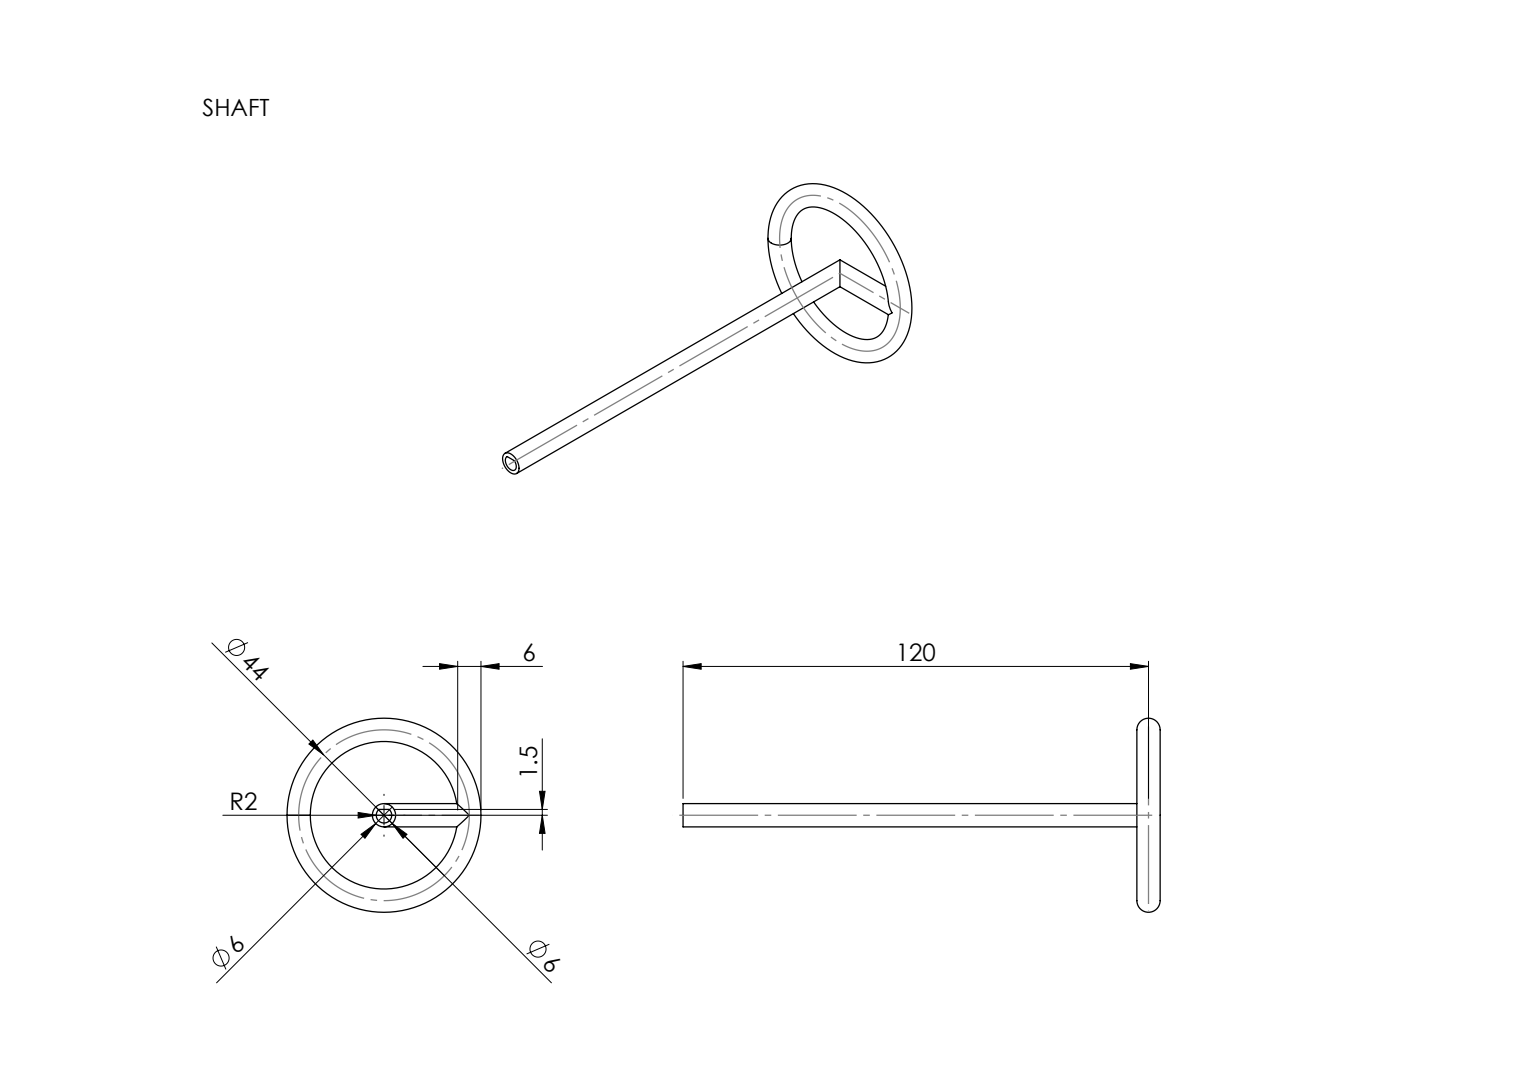
ISO-10303-21;
HEADER;
FILE_DESCRIPTION (('STEP AP214'),
    '1' );
FILE_NAME ('shaft.step',
    '2026-10-08T15:02:10',
    ( '' ),
    ( '' ),
    'SwSTEP 2.0',
    'SolidWorks 2026',
    '' );
FILE_SCHEMA (( 'AUTOMOTIVE_DESIGN' ));
ENDSEC;

DATA;
#29=AXIS2_PLACEMENT_3D ( 'NONE', #18064, #14475, #11199 ) ;
#50=SURFACE_SIDE_STYLE ('',( #17385 ) ) ;
#60=ORIENTED_EDGE ( 'NONE', *, *, #7917, .F. ) ;
#89=CARTESIAN_POINT ( 'NONE',  ( 18.76166303929371537, -3.000000000000002665, -225.0000000000001990 ) ) ;
#116=DIRECTION ( 'NONE',  ( -1.000000000000000000, 0.000000000000000000, 0.000000000000000000 ) ) ;
#168=SURFACE_STYLE_USAGE ( .BOTH. , #50 ) ;
#218=ORIENTED_EDGE ( 'NONE', *, *, #19552, .T. ) ;
#247=CARTESIAN_POINT ( 'NONE',  ( 0.000000000000000000, 0.000000000000000000, -120.0000000000000142 ) ) ;
#414=ORIENTED_EDGE ( 'NONE', *, *, #15901, .T. ) ;
#621=B_SPLINE_CURVE_WITH_KNOTS ( 'NONE', 3,
 ( #8461, #18585, #1249, #11827, #16893, #8123, #21829, #13288, #15329, #18471, #10030, #3033, #3147, #1359, #8232, #15102, #1467, #8343, #15214, #6763, #13633, #22059 ),
 .UNSPECIFIED., .F., .F.,
 ( 4, 2, 2, 2, 2, 2, 2, 2, 2, 2, 4 ),
 ( 0.005800309973860217315, 0.006162931802046735415, 0.006525553630233253515, 0.006888175458419771614, 0.007250797286606289714, 0.007976040942979321577, 0.008701284599352352572, 0.01015177191209841456, 0.01087701556847144729, 0.01123963739665796366, 0.01160225922484448176 ),
 .UNSPECIFIED. ) ;
#691=DIRECTION ( 'NONE',  ( -2.891205793294678696E-17, 0.000000000000000000, -1.000000000000000000 ) ) ;
#722=VERTEX_POINT ( 'NONE', #4541 ) ;
#733=PRODUCT_CONTEXT ( 'NONE', #18778, 'mechanical' ) ;
#748=DIRECTION ( 'NONE',  ( -0.000000000000000000, -1.000000000000000000, 0.000000000000000000 ) ) ;
#799=CARTESIAN_POINT ( 'NONE',  ( 18.92955364685790798, 2.856280672885327832, -224.0526243428037105 ) ) ;
#867=FACE_OUTER_BOUND ( 'NONE', #7455, .T. ) ;
#876=ADVANCED_FACE ( 'NONE', ( #9133 ), #19112, .T. ) ;
#940=DIRECTION ( 'NONE',  ( 1.000000000000000000, 0.000000000000000000, 0.000000000000000000 ) ) ;
#951=CARTESIAN_POINT ( 'NONE',  ( -1.322875655532295136, 1.500000000000000000, -105.0000000000000142 ) ) ;
#991=SHAPE_REPRESENTATION_RELATIONSHIP ( 'NONE' , 'NONE' ,  #6134, #7772 ) ;
#1072=DIRECTION ( 'NONE',  ( -2.891205793294678696E-17, 0.000000000000000000, -1.000000000000000000 ) ) ;
#1087=DIRECTION ( 'NONE',  ( -1.000000000000000000, 0.000000000000000000, 2.891205793294678696E-17 ) ) ;
#1143=AXIS2_PLACEMENT_3D ( 'NONE', #18620, #15780, #13440 ) ;
#1193=CARTESIAN_POINT ( 'NONE',  ( -3.400000000000003908, 0.000000000000000000, -224.9999999999999716 ) ) ;
#1202=ORIENTED_EDGE ( 'NONE', *, *, #20807, .F. ) ;
#1215=CARTESIAN_POINT ( 'NONE',  ( 19.81239090451984097, -2.079411191919079638, -222.8294590615037123 ) ) ;
#1249=CARTESIAN_POINT ( 'NONE',  ( 18.77064933249683065, 2.992341472042430173, -225.2461773443920663 ) ) ;
#1297=DIRECTION ( 'NONE',  ( -2.891205793294678696E-17, 0.000000000000000000, -1.000000000000000000 ) ) ;
#1304=CYLINDRICAL_SURFACE ( 'NONE', #3314, 3.000000000000002665 ) ;
#1319=CARTESIAN_POINT ( 'NONE',  ( -2.775557561562891351E-14, 0.000000000000000000, -105.0000000000000142 ) ) ;
#1327=CARTESIAN_POINT ( 'NONE',  ( 22.00000000000000000, 0.000000000000000000, -221.9999999999999716 ) ) ;
#1359=CARTESIAN_POINT ( 'NONE',  ( 20.28602808787860567, 1.649471991126377768, -227.5337793182429493 ) ) ;
#1463=FACE_OUTER_BOUND ( 'NONE', #17228, .T. ) ;
#1467=CARTESIAN_POINT ( 'NONE',  ( 21.30611872263677498, 0.6836234283288439295, -227.9261315426025760 ) ) ;
#1469=( NAMED_UNIT ( * ) PLANE_ANGLE_UNIT ( ) SI_UNIT ( $, .RADIAN. ) );
#1480=DIRECTION ( 'NONE',  ( -6.123233995736766036E-17, 0.000000000000000000, 1.000000000000000000 ) ) ;
#1549=PLANE ( 'NONE',  #9838 ) ;
#1587=SURFACE_STYLE_FILL_AREA ( #3257 ) ;
#1634=( LENGTH_UNIT ( ) NAMED_UNIT ( * ) SI_UNIT ( .MILLI., .METRE. ) );
#1673=ORIENTED_EDGE ( 'NONE', *, *, #20807, .T. ) ;
#1678=ORIENTED_EDGE ( 'NONE', *, *, #12038, .T. ) ;
#1923=CARTESIAN_POINT ( 'NONE',  ( -3.000000000000034195, 6.000000000000006217, -227.9999999999999716 ) ) ;
#1949=EDGE_CURVE ( 'NONE', #722, #21305, #10868, .T. ) ;
#1961=( GEOMETRIC_REPRESENTATION_CONTEXT ( 3 ) GLOBAL_UNCERTAINTY_ASSIGNED_CONTEXT ( ( #19989 ) ) GLOBAL_UNIT_ASSIGNED_CONTEXT ( ( #1634, #15705, #7260 ) ) REPRESENTATION_CONTEXT ( 'NONE', 'WORKASPACE' ) );
#2075=DIRECTION ( 'NONE',  ( -1.000000000000000000, 0.000000000000000000, 0.000000000000000000 ) ) ;
#2085=CARTESIAN_POINT ( 'NONE',  ( 2.000000000000000000, 0.000000000000000000, -120.0000000000000142 ) ) ;
#2086=ORIENTED_EDGE ( 'NONE', *, *, #21351, .F. ) ;
#2168=CLOSED_SHELL ( 'NONE', ( #876, #15317, #2802, #6387, #3276, #20231, #8918, #6260, #11075, #12311, #16542, #17405, #7759, #13941 ) ) ;
#2200=ORIENTED_EDGE ( 'NONE', *, *, #7776, .F. ) ;
#2204=DIRECTION ( 'NONE',  ( -1.000000000000000000, -1.224646799147353454E-16, 0.000000000000000000 ) ) ;
#2259=AXIS2_PLACEMENT_3D ( 'NONE', #13081, #18367, #16564 ) ;
#2343=DIRECTION ( 'NONE',  ( -1.000000000000000000, 0.000000000000000000, 0.000000000000000000 ) ) ;
#2453=DIRECTION ( 'NONE',  ( 1.000000000000000000, 0.000000000000000000, 0.000000000000000000 ) ) ;
#2484=CARTESIAN_POINT ( 'NONE',  ( 19.66316721362388975, 2.213178807039652973, -222.9648072419893765 ) ) ;
#2565=DIRECTION ( 'NONE',  ( -1.000000000000000000, 0.000000000000000000, 0.000000000000000000 ) ) ;
#2593=FACE_OUTER_BOUND ( 'NONE', #12316, .T. ) ;
#2604=CARTESIAN_POINT ( 'NONE',  ( 1.322875655532295358, 1.500000000000000000, -105.0000000000000142 ) ) ;
#2609=VECTOR ( 'NONE', #2075, 1000.000000000000000 ) ;
#2707=DIRECTION ( 'NONE',  ( 1.000000000000000000, 0.000000000000000000, 0.000000000000000000 ) ) ;
#2762=VERTEX_POINT ( 'NONE', #21336 ) ;
#2802=ADVANCED_FACE ( 'NONE', ( #867 ), #4621, .T. ) ;
#2874=ORIENTED_EDGE ( 'NONE', *, *, #19438, .T. ) ;
#2885=CARTESIAN_POINT ( 'NONE',  ( 19.08116649778970952, -2.725278401796281447, -223.7411956188273621 ) ) ;
#2965=VERTEX_POINT ( 'NONE', #19869 ) ;
#2978=CARTESIAN_POINT ( 'NONE',  ( 22.00000000000000000, 6.162975822039154730E-30, -228.0000000000000000 ) ) ;
#3000=CARTESIAN_POINT ( 'NONE',  ( 19.24993070808567097, -2.578473320807608715, -223.4513235704932299 ) ) ;
#3004=CARTESIAN_POINT ( 'NONE',  ( 21.82657638218437057, -0.1729100361068852398, -227.9962408443968798 ) ) ;
#3033=CARTESIAN_POINT ( 'NONE',  ( 19.66230024959844513, 2.213945732971074332, -227.0341823791074773 ) ) ;
#3102=CARTESIAN_POINT ( 'NONE',  ( 0.000000000000000000, 0.000000000000000000, -120.0000000000000142 ) ) ;
#3147=CARTESIAN_POINT ( 'NONE',  ( 19.81239090451986939, 2.079411191919064983, -227.1705409384963161 ) ) ;
#3190=ORIENTED_EDGE ( 'NONE', *, *, #9938, .T. ) ;
#3194=DIRECTION ( 'NONE',  ( 1.000000000000000000, 0.000000000000000000, 0.000000000000000000 ) ) ;
#3257=FILL_AREA_STYLE ('',( #6873 ) ) ;
#3276=ADVANCED_FACE ( 'NONE', ( #5013 ), #15389, .F. ) ;
#3314=AXIS2_PLACEMENT_3D ( 'NONE', #1193, #18305, #11216 ) ;
#3339=CARTESIAN_POINT ( 'NONE',  ( 19.81538647100171957, -2.076704763782542429, -227.1730004250662773 ) ) ;
#3371=PRESENTATION_STYLE_ASSIGNMENT (( #21940 ) ) ;
#3386=COLOUR_RGB ( '', 0.31764706, 0.68627451, 0.89019608) ;
#3449=CARTESIAN_POINT ( 'NONE',  ( 0.000000000000000000, 0.000000000000000000, -120.0000000000000142 ) ) ;
#3542=ORIENTED_EDGE ( 'NONE', *, *, #3964, .T. ) ;
#3565=EDGE_CURVE ( 'NONE', #8742, #7031, #18647, .T. ) ;
#3572=VERTEX_POINT ( 'NONE', #6600 ) ;
#3663=DIRECTION ( 'NONE',  ( 0.000000000000000000, 0.000000000000000000, -1.000000000000000000 ) ) ;
#3669=CARTESIAN_POINT ( 'NONE',  ( 19.25067847059915849, -2.577822808762990636, -226.5499581033751895 ) ) ;
#3694=DIRECTION ( 'NONE',  ( 1.000000000000000000, 0.000000000000000000, 0.000000000000000000 ) ) ;
#3750=TOROIDAL_SURFACE ( 'NONE', #8452, 22.00000000000000711, 2.999999999999999112 ) ;
#3775=VECTOR ( 'NONE', #17147, 1000.000000000000000 ) ;
#3788=CARTESIAN_POINT ( 'NONE',  ( 18.83061188870375702, -2.941116900365129183, -225.6031553348211958 ) ) ;
#3830=DIRECTION ( 'NONE',  ( 1.000000000000000000, 0.000000000000000000, 0.000000000000000000 ) ) ;
#3964=EDGE_CURVE ( 'NONE', #17015, #11981, #7055, .T. ) ;
#4056=CIRCLE ( 'NONE', #2259, 2.000000000000000000 ) ;
#4072=AXIS2_PLACEMENT_3D ( 'NONE', #9335, #12708, #16635 ) ;
#4111=ORIENTED_EDGE ( 'NONE', *, *, #13596, .T. ) ;
#4126=ORIENTED_EDGE ( 'NONE', *, *, #11026, .T. ) ;
#4175=VECTOR ( 'NONE', #20468, 1000.000000000000000 ) ;
#4250=CYLINDRICAL_SURFACE ( 'NONE', #8056, 3.000000000000002665 ) ;
#4307=ORIENTED_EDGE ( 'NONE', *, *, #10113, .F. ) ;
#4332=FACE_OUTER_BOUND ( 'NONE', #8944, .T. ) ;
#4364=ORIENTED_EDGE ( 'NONE', *, *, #8228, .T. ) ;
#4443=EDGE_CURVE ( 'NONE', #17126, #4726, #6051, .T. ) ;
#4448=ORIENTED_EDGE ( 'NONE', *, *, #14092, .F. ) ;
#4452=ORIENTED_EDGE ( 'NONE', *, *, #1949, .F. ) ;
#4541=CARTESIAN_POINT ( 'NONE',  ( 24.99999999999999645, 3.061616997868383437E-15, -224.9999999999999716 ) ) ;
#4570=ORIENTED_EDGE ( 'NONE', *, *, #14092, .T. ) ;
#4621=TOROIDAL_SURFACE ( 'NONE', #6424, 22.00000000000000711, 2.999999999999999112 ) ;
#4688=CARTESIAN_POINT ( 'NONE',  ( 21.82670294635402897, -0.1727854921979527503, -222.0037445873432205 ) ) ;
#4726=VERTEX_POINT ( 'NONE', #951 ) ;
#4808=DIRECTION ( 'NONE',  ( -0.000000000000000000, -0.000000000000000000, 1.000000000000000000 ) ) ;
#4818=CIRCLE ( 'NONE', #9908, 2.999999999999999112 ) ;
#4840=( NAMED_UNIT ( * ) SI_UNIT ( $, .STERADIAN. ) SOLID_ANGLE_UNIT ( ) );
#4888=CARTESIAN_POINT ( 'NONE',  ( -6.938893903907228378E-15, 0.000000000000000000, -224.9999999999999716 ) ) ;
#5007=EDGE_LOOP ( 'NONE', ( #11084, #5257, #4307, #6425 ) ) ;
#5013=FACE_OUTER_BOUND ( 'NONE', #11808, .T. ) ;
#5025=DIRECTION ( 'NONE',  ( -0.000000000000000000, -0.000000000000000000, 1.000000000000000000 ) ) ;
#5030=CARTESIAN_POINT ( 'NONE',  ( 20.29114891157122358, -1.643118446426441892, -227.5163857825534421 ) ) ;
#5035=ORIENTED_EDGE ( 'NONE', *, *, #17379, .T. ) ;
#5060=( LENGTH_UNIT ( ) NAMED_UNIT ( * ) SI_UNIT ( .MILLI., .METRE. ) );
#5234=ORIENTED_EDGE ( 'NONE', *, *, #19552, .F. ) ;
#5237=LINE ( 'NONE', #13472, #19455 ) ;
#5257=ORIENTED_EDGE ( 'NONE', *, *, #13812, .T. ) ;
#5364=EDGE_LOOP ( 'NONE', ( #11204, #4448, #4126, #60 ) ) ;
#5375=EDGE_CURVE ( 'NONE', #18785, #9979, #5237, .T. ) ;
#5477=CARTESIAN_POINT ( 'NONE',  ( -6.938893903907228378E-15, 0.000000000000000000, -224.9999999999999716 ) ) ;
#5520=FACE_OUTER_BOUND ( 'NONE', #22180, .T. ) ;
#5555=VERTEX_POINT ( 'NONE', #10208 ) ;
#5604=VERTEX_POINT ( 'NONE', #16961 ) ;
#5679=DIRECTION ( 'NONE',  ( -0.000000000000000000, -0.000000000000000000, 1.000000000000000000 ) ) ;
#5701=DIRECTION ( 'NONE',  ( -1.000000000000000000, 0.000000000000000000, 0.000000000000000000 ) ) ;
#5718=CARTESIAN_POINT ( 'NONE',  ( 0.000000000000000000, 0.000000000000000000, -120.0000000000000142 ) ) ;
#5818=CARTESIAN_POINT ( 'NONE',  ( -6.938893903907228378E-15, 0.000000000000000000, -224.9999999999999716 ) ) ;
#5854=AXIS2_PLACEMENT_3D ( 'NONE', #20104, #4808, #20213 ) ;
#5860=CARTESIAN_POINT ( 'NONE',  ( -6.938893903907228378E-15, 0.000000000000000000, -224.9999999999999716 ) ) ;
#5881=ORIENTED_EDGE ( 'NONE', *, *, #3565, .F. ) ;
#5925=ORIENTED_EDGE ( 'NONE', *, *, #8488, .T. ) ;
#5975=AXIS2_PLACEMENT_3D ( 'NONE', #12852, #16554, #20027 ) ;
#6051=CIRCLE ( 'NONE', #19700, 2.000000000000000000 ) ;
#6082=CARTESIAN_POINT ( 'NONE',  ( 19.81538647100178707, 2.076704763782484253, -222.8269995749336658 ) ) ;
#6130=CARTESIAN_POINT ( 'NONE',  ( -22.00000000000001421, 0.000000000000000000, -224.9999999999999716 ) ) ;
#6134=SHAPE_REPRESENTATION ( 'shaft', ( #6677 ), #8503 ) ;
#6240=CIRCLE ( 'NONE', #9120, 2.000000000000000000 ) ;
#6246=DIRECTION ( 'NONE',  ( -2.891205793294678696E-17, 0.000000000000000000, -1.000000000000000000 ) ) ;
#6260=ADVANCED_FACE ( 'NONE', ( #7607, #9625 ), #21757, .T. ) ;
#6325=ORIENTED_EDGE ( 'NONE', *, *, #15901, .F. ) ;
#6327=ORIENTED_EDGE ( 'NONE', *, *, #11715, .T. ) ;
#6383=CARTESIAN_POINT ( 'NONE',  ( 21.56647080447662290, -0.4294288297056042536, -222.0296485764623640 ) ) ;
#6387=ADVANCED_FACE ( 'NONE', ( #5520 ), #12398, .F. ) ;
#6424=AXIS2_PLACEMENT_3D ( 'NONE', #5818, #19543, #1087 ) ;
#6425=ORIENTED_EDGE ( 'NONE', *, *, #11026, .F. ) ;
#6487=DIRECTION ( 'NONE',  ( -1.000000000000000000, 0.000000000000000000, 0.000000000000000000 ) ) ;
#6529=CARTESIAN_POINT ( 'NONE',  ( 2.999999999999972466, -6.000000000000006217, -221.9999999999999716 ) ) ;
#6600=CARTESIAN_POINT ( 'NONE',  ( 22.00000000000000000, 0.000000000000000000, -221.9999999999999716 ) ) ;
#6613=CARTESIAN_POINT ( 'NONE',  ( -2.000000000000000000, 2.449293598294706414E-16, -120.0000000000000142 ) ) ;
#6614=CARTESIAN_POINT ( 'NONE',  ( 19.02965008953347237, -2.769875716686367007, -223.8421603075141491 ) ) ;
#6619=CARTESIAN_POINT ( 'NONE',  ( -2.775557561562891351E-14, 0.000000000000000000, -105.0000000000000142 ) ) ;
#6648=CARTESIAN_POINT ( 'NONE',  ( -3.400000000000003908, 0.000000000000000000, -227.9999999999999716 ) ) ;
#6677=AXIS2_PLACEMENT_3D ( 'NONE', #18028, #16226, #2707 ) ;
#6711=AXIS2_PLACEMENT_3D ( 'NONE', #5860, #691, #14761 ) ;
#6732=CARTESIAN_POINT ( 'NONE',  ( 18.93769218002321253, -2.849225658158391461, -224.0541049803088356 ) ) ;
#6763=CARTESIAN_POINT ( 'NONE',  ( 21.82670294635401831, 0.1727854921979470326, -227.9962554126566943 ) ) ;
#6868=DIRECTION ( 'NONE',  ( -2.891205793294678696E-17, 0.000000000000000000, -1.000000000000000000 ) ) ;
#6873=FILL_AREA_STYLE_COLOUR ( '', #15337 ) ;
#6886=CARTESIAN_POINT ( 'NONE',  ( 2.999999999999970690, 6.000000000000006217, -221.9999999999999716 ) ) ;
#6941=ORIENTED_EDGE ( 'NONE', *, *, #11715, .F. ) ;
#7031=VERTEX_POINT ( 'NONE', #9414 ) ;
#7055=LINE ( 'NONE', #2085, #7143 ) ;
#7143=VECTOR ( 'NONE', #5679, 1000.000000000000000 ) ;
#7260=( NAMED_UNIT ( * ) SI_UNIT ( $, .STERADIAN. ) SOLID_ANGLE_UNIT ( ) );
#7314=CIRCLE ( 'NONE', #16629, 19.00000000000000711 ) ;
#7455=EDGE_LOOP ( 'NONE', ( #14480, #15948, #5925, #2200, #9544 ) ) ;
#7567=EDGE_CURVE ( 'NONE', #7956, #5604, #15692, .T. ) ;
#7607=FACE_BOUND ( 'NONE', #14199, .T. ) ;
#7679=CARTESIAN_POINT ( 'NONE',  ( 18.83061188870378544, 2.941116900365108311, -224.3968446651786337 ) ) ;
#7688=CIRCLE ( 'NONE', #4072, 2.999999999999999112 ) ;
#7715=DIRECTION ( 'NONE',  ( 1.000000000000000000, 0.000000000000000000, 0.000000000000000000 ) ) ;
#7724=ORIENTED_EDGE ( 'NONE', *, *, #21351, .T. ) ;
#7759=ADVANCED_FACE ( 'NONE', ( #2593 ), #7901, .F. ) ;
#7772=ADVANCED_BREP_SHAPE_REPRESENTATION ( '', ( #14254, #6677 ), #8503 ) ;
#7776=EDGE_CURVE ( 'NONE', #3572, #5555, #19145, .T. ) ;
#7793=CARTESIAN_POINT ( 'NONE',  ( 19.38023697009521840, 2.464236985537108904, -223.2772968702357730 ) ) ;
#7795=CARTESIAN_POINT ( 'NONE',  ( -3.000000000000030198, 0.000000000000000000, -105.0000000000000142 ) ) ;
#7817=DIRECTION ( 'NONE',  ( 6.123233995736766036E-17, -0.000000000000000000, -1.000000000000000000 ) ) ;
#7896=EDGE_LOOP ( 'NONE', ( #4570, #14262 ) ) ;
#7901=PLANE ( 'NONE',  #5975 ) ;
#7917=EDGE_CURVE ( 'NONE', #2965, #2762, #20795, .T. ) ;
#7956=VERTEX_POINT ( 'NONE', #20244 ) ;
#7975=FACE_OUTER_BOUND ( 'NONE', #19124, .T. ) ;
#8009=CARTESIAN_POINT ( 'NONE',  ( 21.30903826138442270, 0.6807850236355362794, -222.0732863424555035 ) ) ;
#8056=AXIS2_PLACEMENT_3D ( 'NONE', #18326, #2453, #14732 ) ;
#8085=UNCERTAINTY_MEASURE_WITH_UNIT (LENGTH_MEASURE( 1.000000000000000082E-05 ), #5060, 'distance_accuracy_value', 'NONE');
#8090=CARTESIAN_POINT ( 'NONE',  ( 21.30611872263680695, -0.6836234283288118441, -222.0738684573972819 ) ) ;
#8111=VECTOR ( 'NONE', #3694, 1000.000000000000000 ) ;
#8123=CARTESIAN_POINT ( 'NONE',  ( 18.89697753402894875, 2.884212079946345320, -225.8338386031039988 ) ) ;
#8149=CARTESIAN_POINT ( 'NONE',  ( -25.00000000000001066, 0.000000000000000000, -224.9999999999999716 ) ) ;
#8177=EDGE_CURVE ( 'NONE', #5555, #9014, #621, .T. ) ;
#8198=CARTESIAN_POINT ( 'NONE',  ( 2.000000000000000000, 0.000000000000000000, -120.0000000000000142 ) ) ;
#8228=EDGE_CURVE ( 'NONE', #2762, #9014, #20357, .T. ) ;
#8232=CARTESIAN_POINT ( 'NONE',  ( 20.61940245508341363, 1.339931705218432079, -227.7063352817440318 ) ) ;
#8234=( NAMED_UNIT ( * ) PLANE_ANGLE_UNIT ( ) SI_UNIT ( $, .RADIAN. ) );
#8259=LINE ( 'NONE', #16921, #3775 ) ;
#8288=EDGE_CURVE ( 'NONE', #5604, #21305, #10669, .T. ) ;
#8302=DIRECTION ( 'NONE',  ( -2.891205793294678696E-17, 0.000000000000000000, -1.000000000000000000 ) ) ;
#8343=CARTESIAN_POINT ( 'NONE',  ( 21.56647080447661224, 0.4294288297056144676, -227.9703514235376076 ) ) ;
#8413=ORIENTED_EDGE ( 'NONE', *, *, #1949, .T. ) ;
#8430=FACE_OUTER_BOUND ( 'NONE', #19282, .T. ) ;
#8452=AXIS2_PLACEMENT_3D ( 'NONE', #4888, #1072, #19966 ) ;
#8461=CARTESIAN_POINT ( 'NONE',  ( 18.76166303929371537, 3.000000000000002665, -224.9999999999997442 ) ) ;
#8488=EDGE_CURVE ( 'NONE', #5604, #5555, #7314, .T. ) ;
#8503=( GEOMETRIC_REPRESENTATION_CONTEXT ( 3 ) GLOBAL_UNCERTAINTY_ASSIGNED_CONTEXT ( ( #8085 ) ) GLOBAL_UNIT_ASSIGNED_CONTEXT ( ( #5060, #1469, #11937 ) ) REPRESENTATION_CONTEXT ( 'NONE', 'WORKASPACE' ) );
#8742=VERTEX_POINT ( 'NONE', #12799 ) ;
#8918=ADVANCED_FACE ( 'NONE', ( #4332 ), #1304, .T. ) ;
#8944=EDGE_LOOP ( 'NONE', ( #12143, #414, #16206, #20787, #17415 ) ) ;
#9014=VERTEX_POINT ( 'NONE', #2978 ) ;
#9120=AXIS2_PLACEMENT_3D ( 'NONE', #5718, #19114, #2343 ) ;
#9133=FACE_OUTER_BOUND ( 'NONE', #18914, .T. ) ;
#9165=ORIENTED_EDGE ( 'NONE', *, *, #4443, .F. ) ;
#9335=CARTESIAN_POINT ( 'NONE',  ( 22.00000000000000000, 2.694222958124177598E-15, -224.9999999999999716 ) ) ;
#9414=CARTESIAN_POINT ( 'NONE',  ( -1.322875655532295136, 1.500000000000000000, -120.0000000000000142 ) ) ;
#9476=CARTESIAN_POINT ( 'NONE',  ( 20.12875910279714020, 1.792218354162522953, -222.5869962921167655 ) ) ;
#9544=ORIENTED_EDGE ( 'NONE', *, *, #13072, .T. ) ;
#9568=ORIENTED_EDGE ( 'NONE', *, *, #12948, .F. ) ;
#9625=FACE_OUTER_BOUND ( 'NONE', #7896, .T. ) ;
#9695=LINE ( 'NONE', #7795, #19957 ) ;
#9838=AXIS2_PLACEMENT_3D ( 'NONE', #3449, #3663, #17191 ) ;
#9883=CARTESIAN_POINT ( 'NONE',  ( 19.66230024959842382, -2.213945732971099201, -222.9658176208924942 ) ) ;
#9887=CARTESIAN_POINT ( 'NONE',  ( 21.30903826138435875, -0.6807850236355832418, -227.9267136575444397 ) ) ;
#9891=TOROIDAL_SURFACE ( 'NONE', #12418, 22.00000000000000711, 2.999999999999999112 ) ;
#9908=AXIS2_PLACEMENT_3D ( 'NONE', #12017, #12353, #2204 ) ;
#9938=EDGE_CURVE ( 'NONE', #9979, #11981, #4056, .T. ) ;
#9979=VERTEX_POINT ( 'NONE', #2604 ) ;
#9998=CARTESIAN_POINT ( 'NONE',  ( 18.77064933249684486, -2.992341472042426620, -224.7538226556079337 ) ) ;
#10030=CARTESIAN_POINT ( 'NONE',  ( 19.38184807124233799, 2.462809743167411636, -226.7245352501389846 ) ) ;
#10031=( BOUNDED_CURVE ( )  B_SPLINE_CURVE ( 3, ( #21949, #1923, #6886, #10480 ),
 .UNSPECIFIED., .F., .F. ) 
 B_SPLINE_CURVE_WITH_KNOTS ( ( 4, 4 ),
 ( 0.000000000000000000, 3.141592653589793116 ),
 .UNSPECIFIED. ) 
 CURVE ( )  GEOMETRIC_REPRESENTATION_ITEM ( )  RATIONAL_B_SPLINE_CURVE ( ( 1.000000000000000000, 0.3333333333333333703, 0.3333333333333333703, 1.000000000000000000 ) ) 
 REPRESENTATION_ITEM ( '' )  );
#10043=CARTESIAN_POINT ( 'NONE',  ( -2.775557561562891351E-14, 0.000000000000000000, -105.0000000000000142 ) ) ;
#10087=ORIENTED_EDGE ( 'NONE', *, *, #13361, .F. ) ;
#10105=LINE ( 'NONE', #6613, #19527 ) ;
#10110=CARTESIAN_POINT ( 'NONE',  ( 20.79630060232303634, -1.171431775223993110, -227.7672307301629075 ) ) ;
#10113=EDGE_CURVE ( 'NONE', #2762, #2965, #10031, .T. ) ;
#10159=VECTOR ( 'NONE', #116, 1000.000000000000000 ) ;
#10208=CARTESIAN_POINT ( 'NONE',  ( 18.76166303929371537, 3.000000000000002665, -224.9999999999997442 ) ) ;
#10266=CIRCLE ( 'NONE', #18887, 2.000000000000000000 ) ;
#10268=DIRECTION ( 'NONE',  ( -0.000000000000000000, -0.000000000000000000, 1.000000000000000000 ) ) ;
#10301=FILL_AREA_STYLE ('',( #14131 ) ) ;
#10455=ORIENTED_EDGE ( 'NONE', *, *, #4443, .T. ) ;
#10480=CARTESIAN_POINT ( 'NONE',  ( 2.999999999999971578, 3.673940397442062826E-16, -221.9999999999999716 ) ) ;
#10523=CYLINDRICAL_SURFACE ( 'NONE', #14143, 3.000000000000002665 ) ;
#10571=EDGE_CURVE ( 'NONE', #15054, #11155, #20224, .T. ) ;
#10669=CIRCLE ( 'NONE', #19625, 3.000000000000002665 ) ;
#10868=CIRCLE ( 'NONE', #17702, 25.00000000000000355 ) ;
#10884=CARTESIAN_POINT ( 'NONE',  ( -22.00000000000001421, 0.000000000000000000, -224.9999999999999716 ) ) ;
#10931=CIRCLE ( 'NONE', #17414, 25.00000000000000355 ) ;
#11026=EDGE_CURVE ( 'NONE', #11155, #2762, #9695, .T. ) ;
#11075=ADVANCED_FACE ( 'NONE', ( #13249 ), #16516, .T. ) ;
#11084=ORIENTED_EDGE ( 'NONE', *, *, #10571, .F. ) ;
#11155=VERTEX_POINT ( 'NONE', #16963 ) ;
#11189=ORIENTED_EDGE ( 'NONE', *, *, #8488, .F. ) ;
#11199=DIRECTION ( 'NONE',  ( 1.000000000000000000, 0.000000000000000000, 6.123233995736766036E-17 ) ) ;
#11204=ORIENTED_EDGE ( 'NONE', *, *, #13812, .F. ) ;
#11216=DIRECTION ( 'NONE',  ( 0.000000000000000000, 0.000000000000000000, -1.000000000000000000 ) ) ;
#11270=CARTESIAN_POINT ( 'NONE',  ( 18.76166303929373314, 2.999999999999994227, -224.8778586954795742 ) ) ;
#11320=DIRECTION ( 'NONE',  ( -0.000000000000000000, -1.000000000000000000, 0.000000000000000000 ) ) ;
#11372=MECHANICAL_DESIGN_GEOMETRIC_PRESENTATION_REPRESENTATION('',(#21055),#12454);
#11439=ORIENTED_EDGE ( 'NONE', *, *, #3565, .T. ) ;
#11452=UNCERTAINTY_MEASURE_WITH_UNIT (LENGTH_MEASURE( 1.000000000000000082E-05 ), #17010, 'distance_accuracy_value', 'NONE');
#11456=CARTESIAN_POINT ( 'NONE',  ( 18.83090365933348664, -2.940867245730338642, -224.3956276138626720 ) ) ;
#11550=DIRECTION ( 'NONE',  ( 0.000000000000000000, 0.000000000000000000, -1.000000000000000000 ) ) ;
#11593=DIRECTION ( 'NONE',  ( -1.000000000000000000, 0.000000000000000000, 2.891205793294678696E-17 ) ) ;
#11594=CARTESIAN_POINT ( 'NONE',  ( 1.322875655532295136, 1.500000000000000000, -120.0000000000000142 ) ) ;
#11601=SURFACE_SIDE_STYLE ('',( #1587 ) ) ;
#11659=ORIENTED_EDGE ( 'NONE', *, *, #5375, .T. ) ;
#11669=MECHANICAL_DESIGN_GEOMETRIC_PRESENTATION_REPRESENTATION('',(#19924),#1961);
#11672=PRODUCT_DEFINITION_CONTEXT ( 'detailed design', #15204, 'design' ) ;
#11690=ORIENTED_EDGE ( 'NONE', *, *, #8288, .T. ) ;
#11715=EDGE_CURVE ( 'NONE', #17015, #8742, #6240, .T. ) ;
#11778=ORIENTED_EDGE ( 'NONE', *, *, #12038, .F. ) ;
#11808=EDGE_LOOP ( 'NONE', ( #218, #3542, #21945, #15473 ) ) ;
#11827=CARTESIAN_POINT ( 'NONE',  ( 18.80535572547204026, 2.962702208451975849, -225.4869357187871231 ) ) ;
#11884=ORIENTED_EDGE ( 'NONE', *, *, #21643, .F. ) ;
#11902=CARTESIAN_POINT ( 'NONE',  ( 20.61940245508336034, -1.339931705218483815, -222.2936647182560819 ) ) ;
#11937=( NAMED_UNIT ( * ) SI_UNIT ( $, .STERADIAN. ) SOLID_ANGLE_UNIT ( ) );
#11957=EDGE_LOOP ( 'NONE', ( #4452, #14287, #9568, #20145, #11690 ) ) ;
#11981=VERTEX_POINT ( 'NONE', #15866 ) ;
#12017=CARTESIAN_POINT ( 'NONE',  ( 22.00000000000000000, 2.694222958124177598E-15, -224.9999999999999716 ) ) ;
#12038=EDGE_CURVE ( 'NONE', #722, #9014, #7688, .T. ) ;
#12118=DIRECTION ( 'NONE',  ( 0.000000000000000000, 0.000000000000000000, 1.000000000000000000 ) ) ;
#12143=ORIENTED_EDGE ( 'NONE', *, *, #10113, .T. ) ;
#12311=ADVANCED_FACE ( 'NONE', ( #7975 ), #4250, .T. ) ;
#12316=EDGE_LOOP ( 'NONE', ( #11659, #2874, #11884, #1202 ) ) ;
#12353=DIRECTION ( 'NONE',  ( -1.224646799147353207E-16, 1.000000000000000000, 3.540705920434612608E-33 ) ) ;
#12357=CARTESIAN_POINT ( 'NONE',  ( 18.77038210872051849, -2.992569296362960873, -225.2431827457303655 ) ) ;
#12398=CYLINDRICAL_SURFACE ( 'NONE', #19604, 2.000000000000000000 ) ;
#12418=AXIS2_PLACEMENT_3D ( 'NONE', #22265, #6868, #11593 ) ;
#12428=ORIENTED_EDGE ( 'NONE', *, *, #13361, .T. ) ;
#12435=PRESENTATION_STYLE_ASSIGNMENT (( #168 ) ) ;
#12454=( GEOMETRIC_REPRESENTATION_CONTEXT ( 3 ) GLOBAL_UNCERTAINTY_ASSIGNED_CONTEXT ( ( #11452 ) ) GLOBAL_UNIT_ASSIGNED_CONTEXT ( ( #17010, #8234, #4840 ) ) REPRESENTATION_CONTEXT ( 'NONE', 'WORKASPACE' ) );
#12473=CARTESIAN_POINT ( 'NONE',  ( 18.80464855560517989, -2.963306505625492804, -225.4831391053028824 ) ) ;
#12527=AXIS2_PLACEMENT_3D ( 'NONE', #15053, #11550, #16846 ) ;
#12708=DIRECTION ( 'NONE',  ( -1.224646799147353207E-16, 1.000000000000000000, 3.540705920434612608E-33 ) ) ;
#12741=CARTESIAN_POINT ( 'NONE',  ( 22.00000000000000000, 0.000000000000000000, -221.9999999999999716 ) ) ;
#12777=DIRECTION ( 'NONE',  ( 6.123233995736766036E-17, -0.000000000000000000, -1.000000000000000000 ) ) ;
#12799=CARTESIAN_POINT ( 'NONE',  ( -2.000000000000000000, 2.449293598294706414E-16, -120.0000000000000142 ) ) ;
#12852=CARTESIAN_POINT ( 'NONE',  ( 1.322875655532295358, 1.500000000000000000, -378.2244600276337678 ) ) ;
#12890=SHAPE_DEFINITION_REPRESENTATION ( #20353, #6134 ) ;
#12948=EDGE_CURVE ( 'NONE', #7956, #3572, #13175, .T. ) ;
#12957=CARTESIAN_POINT ( 'NONE',  ( 19.02418198972967289, 2.774848290581965582, -223.8390704070222910 ) ) ;
#13040=CARTESIAN_POINT ( 'NONE',  ( 0.000000000000000000, 0.000000000000000000, -120.0000000000000142 ) ) ;
#13072=EDGE_CURVE ( 'NONE', #3572, #722, #4818, .T. ) ;
#13080=AXIS2_PLACEMENT_3D ( 'NONE', #1319, #8302, #6487 ) ;
#13081=CARTESIAN_POINT ( 'NONE',  ( 0.000000000000000000, 0.000000000000000000, -105.0000000000000142 ) ) ;
#13175=B_SPLINE_CURVE_WITH_KNOTS ( 'NONE', 3,
 ( #20209, #21797, #9998, #15177, #11456, #15293, #6732, #6614, #2885, #3000, #20099, #9883, #1215, #18767, #11902, #18663, #8090, #6383, #20437, #4688, #16747, #1327 ),
 .UNSPECIFIED., .F., .F.,
 ( 4, 2, 2, 2, 2, 2, 2, 2, 2, 2, 4 ),
 ( 0.005800309973861407335, 0.006162931802048039927, 0.006525553630234673386, 0.006888175458421305977, 0.007250797286607938569, 0.007976040942981144771, 0.008701284599354350974, 0.01015177191210072175, 0.01087701556847389672, 0.01123963739666048595, 0.01160225922484707343 ),
 .UNSPECIFIED. ) ;
#13184=CARTESIAN_POINT ( 'NONE',  ( 21.65362371779454520, 0.3438195010044668432, -222.0185330407754520 ) ) ;
#13249=FACE_OUTER_BOUND ( 'NONE', #5364, .T. ) ;
#13288=CARTESIAN_POINT ( 'NONE',  ( 19.02965008953349368, 2.769875716686356348, -226.1578396924859078 ) ) ;
#13361=EDGE_CURVE ( 'NONE', #21305, #5604, #18535, .T. ) ;
#13399=CARTESIAN_POINT ( 'NONE',  ( -3.000000000000034195, -6.000000000000006217, -227.9999999999999716 ) ) ;
#13440=DIRECTION ( 'NONE',  ( -1.000000000000000000, 0.000000000000000000, 2.891205793294678696E-17 ) ) ;
#13472=CARTESIAN_POINT ( 'NONE',  ( 1.322875655532295358, 1.500000000000000000, -378.2244600276337678 ) ) ;
#13534=PRODUCT_DEFINITION_FORMATION_WITH_SPECIFIED_SOURCE ( 'ANY', '', #16780, .NOT_KNOWN. ) ;
#13596=EDGE_CURVE ( 'NONE', #21305, #722, #10931, .T. ) ;
#13604=CARTESIAN_POINT ( 'NONE',  ( 22.00000000000000000, 6.162975822039154730E-30, -228.0000000000000000 ) ) ;
#13609=ORIENTED_EDGE ( 'NONE', *, *, #3964, .F. ) ;
#13633=CARTESIAN_POINT ( 'NONE',  ( 21.91452165549922881, 0.08546329518220173449, -228.0000000000000853 ) ) ;
#13713=CYLINDRICAL_SURFACE ( 'NONE', #5854, 2.000000000000000000 ) ;
#13800=DIRECTION ( 'NONE',  ( -2.891205793294678696E-17, 0.000000000000000000, -1.000000000000000000 ) ) ;
#13812=EDGE_CURVE ( 'NONE', #15054, #2965, #20293, .T. ) ;
#13916=DIRECTION ( 'NONE',  ( -1.000000000000000000, 0.000000000000000000, 0.000000000000000000 ) ) ;
#13941=ADVANCED_FACE ( 'NONE', ( #16495 ), #3750, .T. ) ;
#13964=CARTESIAN_POINT ( 'NONE',  ( -3.400000000000003908, 3.673940397442062826E-16, -221.9999999999999716 ) ) ;
#14092=EDGE_CURVE ( 'NONE', #11155, #15054, #18846, .T. ) ;
#14131=FILL_AREA_STYLE_COLOUR ( '', #3386 ) ;
#14143=AXIS2_PLACEMENT_3D ( 'NONE', #6619, #13800, #13916 ) ;
#14155=B_SPLINE_CURVE_WITH_KNOTS ( 'NONE', 3,
 ( #13604, #20328, #3004, #22147, #18667, #9887, #16753, #10110, #20441, #5030, #18771, #3339, #17090, #15508, #3669, #21002, #20776, #3788, #12473, #12357, #19207, #89 ),
 .UNSPECIFIED., .F., .F.,
 ( 4, 2, 2, 2, 2, 2, 2, 2, 2, 2, 4 ),
 ( -1.095445575531460033E-05, 0.0003522495710957299596, 0.0007154535979467744602, 0.001441861651648853378, 0.002168269705350933489, 0.002894677759053012733, 0.003621085812755091976, 0.004347493866457172521, 0.005073901920159251330, 0.005437105947010329766, 0.005800309973861407335 ),
 .UNSPECIFIED. ) ;
#14199=EDGE_LOOP ( 'NONE', ( #15419, #3190, #7724, #10455 ) ) ;
#14254=MANIFOLD_SOLID_BREP ( 'Sweep2', #2168 ) ;
#14262=ORIENTED_EDGE ( 'NONE', *, *, #10571, .T. ) ;
#14287=ORIENTED_EDGE ( 'NONE', *, *, #13072, .F. ) ;
#14346=ORIENTED_EDGE ( 'NONE', *, *, #8177, .F. ) ;
#14434=CARTESIAN_POINT ( 'NONE',  ( 20.62542899963660759, 1.332263963074341584, -222.3060979289667216 ) ) ;
#14460=CARTESIAN_POINT ( 'NONE',  ( 1.322875655532295358, 1.500000000000000000, -120.0000000000000000 ) ) ;
#14475=DIRECTION ( 'NONE',  ( -6.123233995736766036E-17, 0.000000000000000000, 1.000000000000000000 ) ) ;
#14480=ORIENTED_EDGE ( 'NONE', *, *, #13596, .F. ) ;
#14658=CARTESIAN_POINT ( 'NONE',  ( 21.56733749965854940, 0.4285765077750016694, -222.0295450773661230 ) ) ;
#14732=DIRECTION ( 'NONE',  ( 0.000000000000000000, 0.000000000000000000, -1.000000000000000000 ) ) ;
#14761=DIRECTION ( 'NONE',  ( -1.000000000000000000, 0.000000000000000000, 0.000000000000000000 ) ) ;
#14876=CARTESIAN_POINT ( 'NONE',  ( 21.91438441782059954, 0.08560050869924538952, -222.0000000000000000 ) ) ;
#15053=CARTESIAN_POINT ( 'NONE',  ( 0.000000000000000000, 0.000000000000000000, -120.0000000000000142 ) ) ;
#15054=VERTEX_POINT ( 'NONE', #20576 ) ;
#15102=CARTESIAN_POINT ( 'NONE',  ( 21.13193872423781272, 0.8515989525826543893, -227.8817869685189237 ) ) ;
#15147=DIRECTION ( 'NONE',  ( -1.000000000000000000, 0.000000000000000000, 0.000000000000000000 ) ) ;
#15177=CARTESIAN_POINT ( 'NONE',  ( 18.80535572547204382, -2.962702208451977626, -224.5130642812128485 ) ) ;
#15204=APPLICATION_CONTEXT ( 'automotive_design' ) ;
#15214=CARTESIAN_POINT ( 'NONE',  ( 21.65323058444409199, 0.3442074641359742504, -227.9814296144337220 ) ) ;
#15293=CARTESIAN_POINT ( 'NONE',  ( 18.89697753402895586, -2.884212079946346652, -224.1661613968960864 ) ) ;
#15311=ORIENTED_EDGE ( 'NONE', *, *, #16633, .T. ) ;
#15317=ADVANCED_FACE ( 'NONE', ( #1463 ), #9891, .T. ) ;
#15329=CARTESIAN_POINT ( 'NONE',  ( 19.08116649778970952, 2.725278401796274341, -226.2588043811726379 ) ) ;
#15337=COLOUR_RGB ( '', 0.31764706, 0.68627451, 0.89019608) ;
#15389=CYLINDRICAL_SURFACE ( 'NONE', #16487, 2.000000000000000000 ) ;
#15419=ORIENTED_EDGE ( 'NONE', *, *, #19438, .F. ) ;
#15473=ORIENTED_EDGE ( 'NONE', *, *, #5375, .F. ) ;
#15508=CARTESIAN_POINT ( 'NONE',  ( 19.38023697009515800, -2.464236985537147095, -226.7227031297641986 ) ) ;
#15692=CIRCLE ( 'NONE', #6711, 19.00000000000000711 ) ;
#15705=( NAMED_UNIT ( * ) PLANE_ANGLE_UNIT ( ) SI_UNIT ( $, .RADIAN. ) );
#15780=DIRECTION ( 'NONE',  ( -2.891205793294678696E-17, 0.000000000000000000, -1.000000000000000000 ) ) ;
#15866=CARTESIAN_POINT ( 'NONE',  ( 2.000000000000000000, 0.000000000000000000, -105.0000000000000142 ) ) ;
#15901=EDGE_CURVE ( 'NONE', #2965, #3572, #19117, .T. ) ;
#15928=LINE ( 'NONE', #14460, #2609 ) ;
#15948=ORIENTED_EDGE ( 'NONE', *, *, #8288, .F. ) ;
#16206=ORIENTED_EDGE ( 'NONE', *, *, #7776, .T. ) ;
#16224=CARTESIAN_POINT ( 'NONE',  ( 21.82657638218438478, 0.1729100361068894309, -222.0037591556030918 ) ) ;
#16226=DIRECTION ( 'NONE',  ( 0.000000000000000000, 0.000000000000000000, 1.000000000000000000 ) ) ;
#16317=ORIENTED_EDGE ( 'NONE', *, *, #12948, .T. ) ;
#16346=PRODUCT_DEFINITION ( 'UNKNOWN', '', #13534, #11672 ) ;
#16386=DIRECTION ( 'NONE',  ( 0.000000000000000000, 0.000000000000000000, -1.000000000000000000 ) ) ;
#16487=AXIS2_PLACEMENT_3D ( 'NONE', #3102, #16734, #20088 ) ;
#16495=FACE_OUTER_BOUND ( 'NONE', #11957, .T. ) ;
#16516=CYLINDRICAL_SURFACE ( 'NONE', #13080, 3.000000000000002665 ) ;
#16542=ADVANCED_FACE ( 'NONE', ( #8430 ), #13713, .F. ) ;
#16554=DIRECTION ( 'NONE',  ( 0.000000000000000000, 1.000000000000000000, -0.000000000000000000 ) ) ;
#16564=DIRECTION ( 'NONE',  ( 1.000000000000000000, -3.552713678800500929E-15, 0.000000000000000000 ) ) ;
#16629=AXIS2_PLACEMENT_3D ( 'NONE', #5477, #21328, #5701 ) ;
#16633=EDGE_CURVE ( 'NONE', #9014, #7956, #14155, .T. ) ;
#16635=DIRECTION ( 'NONE',  ( -1.000000000000000000, -1.224646799147353454E-16, 0.000000000000000000 ) ) ;
#16648=AXIS2_PLACEMENT_3D ( 'NONE', #10043, #1480, #20710 ) ;
#16734=DIRECTION ( 'NONE',  ( -0.000000000000000000, -0.000000000000000000, 1.000000000000000000 ) ) ;
#16747=CARTESIAN_POINT ( 'NONE',  ( 21.91452165549967290, -0.08546329518268500069, -222.0000000000000000 ) ) ;
#16753=CARTESIAN_POINT ( 'NONE',  ( 21.13757381859892348, -0.8461838617117842798, -227.8833645607415974 ) ) ;
#16780=PRODUCT ( 'shaft', 'shaft', '', ( #733 ) ) ;
#16846=DIRECTION ( 'NONE',  ( -1.000000000000000000, 0.000000000000000000, 0.000000000000000000 ) ) ;
#16875=DIRECTION ( 'NONE',  ( -2.891205793294678696E-17, 0.000000000000000000, -1.000000000000000000 ) ) ;
#16893=CARTESIAN_POINT ( 'NONE',  ( 18.83090365933349020, 2.940867245730331980, -225.6043723861373280 ) ) ;
#16921=CARTESIAN_POINT ( 'NONE',  ( -1.322875655532295358, 1.500000000000000000, -378.2244600276337678 ) ) ;
#16961=CARTESIAN_POINT ( 'NONE',  ( -19.00000000000001421, 0.000000000000000000, -224.9999999999999716 ) ) ;
#16963=CARTESIAN_POINT ( 'NONE',  ( -3.000000000000030198, 0.000000000000000000, -105.0000000000000142 ) ) ;
#17010=( LENGTH_UNIT ( ) NAMED_UNIT ( * ) SI_UNIT ( .MILLI., .METRE. ) );
#17015=VERTEX_POINT ( 'NONE', #8198 ) ;
#17076=AXIS2_PLACEMENT_3D ( 'NONE', #18407, #18632, #3194 ) ;
#17090=CARTESIAN_POINT ( 'NONE',  ( 19.66316721362375475, -2.213178807039759111, -227.0351927580104814 ) ) ;
#17101=DIRECTION ( 'NONE',  ( -1.000000000000000000, 0.000000000000000000, 0.000000000000000000 ) ) ;
#17126=VERTEX_POINT ( 'NONE', #20321 ) ;
#17147=DIRECTION ( 'NONE',  ( 0.000000000000000000, 0.000000000000000000, 1.000000000000000000 ) ) ;
#17191=DIRECTION ( 'NONE',  ( -1.000000000000000000, 0.000000000000000000, -0.000000000000000000 ) ) ;
#17228=EDGE_LOOP ( 'NONE', ( #10087, #4111, #1678, #14346, #11189 ) ) ;
#17379=EDGE_CURVE ( 'NONE', #8742, #17126, #10105, .T. ) ;
#17385=SURFACE_STYLE_FILL_AREA ( #10301 ) ;
#17405=ADVANCED_FACE ( 'NONE', ( #18765 ), #1549, .F. ) ;
#17414=AXIS2_PLACEMENT_3D ( 'NONE', #20074, #1297, #15147 ) ;
#17415=ORIENTED_EDGE ( 'NONE', *, *, #8228, .F. ) ;
#17426=CARTESIAN_POINT ( 'NONE',  ( -3.000000000000033751, 0.000000000000000000, -227.9999999999999716 ) ) ;
#17458=ORIENTED_EDGE ( 'NONE', *, *, #16633, .F. ) ;
#17702=AXIS2_PLACEMENT_3D ( 'NONE', #22261, #16875, #17101 ) ;
#17712=AXIS2_PLACEMENT_3D ( 'NONE', #13040, #17784, #2565 ) ;
#17784=DIRECTION ( 'NONE',  ( 0.000000000000000000, 0.000000000000000000, -1.000000000000000000 ) ) ;
#17919=CARTESIAN_POINT ( 'NONE',  ( 20.29114891157137635, 1.643118446426296675, -222.4836142174464726 ) ) ;
#18028=CARTESIAN_POINT ( 'NONE',  ( 0.000000000000000000, 0.000000000000000000, 0.000000000000000000 ) ) ;
#18064=CARTESIAN_POINT ( 'NONE',  ( -2.775557561562891351E-14, 0.000000000000000000, -105.0000000000000142 ) ) ;
#18139=CARTESIAN_POINT ( 'NONE',  ( 18.76166303929371537, 3.000000000000002665, -224.9999999999997442 ) ) ;
#18298=CARTESIAN_POINT ( 'NONE',  ( 2.999999999999975131, 3.673940397442062826E-16, -105.0000000000000142 ) ) ;
#18305=DIRECTION ( 'NONE',  ( 1.000000000000000000, 0.000000000000000000, 0.000000000000000000 ) ) ;
#18326=CARTESIAN_POINT ( 'NONE',  ( -3.400000000000003908, 0.000000000000000000, -224.9999999999999716 ) ) ;
#18367=DIRECTION ( 'NONE',  ( 6.123233995736766036E-17, -0.000000000000000000, -1.000000000000000000 ) ) ;
#18407=CARTESIAN_POINT ( 'NONE',  ( -2.775557561562891351E-14, 0.000000000000000000, -105.0000000000000142 ) ) ;
#18471=CARTESIAN_POINT ( 'NONE',  ( 19.24993070808566387, 2.578473320807614488, -226.5486764295067417 ) ) ;
#18535=CIRCLE ( 'NONE', #20993, 3.000000000000002665 ) ;
#18585=CARTESIAN_POINT ( 'NONE',  ( 18.76166303929370827, 3.000000000000011990, -225.1219455178571707 ) ) ;
#18620=CARTESIAN_POINT ( 'NONE',  ( -6.938893903907228378E-15, 0.000000000000000000, -224.9999999999999716 ) ) ;
#18632=DIRECTION ( 'NONE',  ( -6.123233995736766036E-17, 0.000000000000000000, 1.000000000000000000 ) ) ;
#18647=CIRCLE ( 'NONE', #12527, 2.000000000000000000 ) ;
#18663=CARTESIAN_POINT ( 'NONE',  ( 21.13193872423781627, -0.8515989525826406226, -222.1182130314809910 ) ) ;
#18667=CARTESIAN_POINT ( 'NONE',  ( 21.56733749965853164, -0.4285765077750153251, -227.9704549226337917 ) ) ;
#18765=FACE_OUTER_BOUND ( 'NONE', #21123, .T. ) ;
#18767=CARTESIAN_POINT ( 'NONE',  ( 20.28602808787868739, -1.649471991126303827, -222.4662206817569370 ) ) ;
#18771=CARTESIAN_POINT ( 'NONE',  ( 20.12875910279704073, -1.792218354162612881, -227.4130037078831776 ) ) ;
#18778=APPLICATION_CONTEXT ( 'automotive_design' ) ;
#18785=VERTEX_POINT ( 'NONE', #11594 ) ;
#18846=CIRCLE ( 'NONE', #17076, 3.000000000000002665 ) ;
#18887=AXIS2_PLACEMENT_3D ( 'NONE', #21854, #7817, #940 ) ;
#18914=EDGE_LOOP ( 'NONE', ( #11778, #8413, #12428, #19654, #17458 ) ) ;
#19112=TOROIDAL_SURFACE ( 'NONE', #1143, 22.00000000000000711, 2.999999999999999112 ) ;
#19114=DIRECTION ( 'NONE',  ( 0.000000000000000000, 0.000000000000000000, -1.000000000000000000 ) ) ;
#19117=LINE ( 'NONE', #13964, #8111 ) ;
#19124=EDGE_LOOP ( 'NONE', ( #6325, #20980, #4364, #15311, #16317 ) ) ;
#19145=B_SPLINE_CURVE_WITH_KNOTS ( 'NONE', 3,
 ( #12741, #14876, #16224, #13184, #14658, #8009, #21385, #19586, #14434, #17919, #9476, #6082, #2484, #7793, #21601, #12957, #799, #7679, #19801, #19694, #11270, #18139 ),
 .UNSPECIFIED., .F., .F.,
 ( 4, 2, 2, 2, 2, 2, 2, 2, 2, 2, 4 ),
 ( -1.095445575531557103E-05, 0.0003522495710956626848, 0.0007154535979466409949, 0.001441861651648580159, 0.002168269705350519324, 0.002894677759052458055, 0.003621085812754397219, 0.004347493866456335516, 0.005073901920158274681, 0.005437105947009245564, 0.005800309973860217315 ),
 .UNSPECIFIED. ) ;
#19198=VECTOR ( 'NONE', #6246, 1000.000000000000000 ) ;
#19207=CARTESIAN_POINT ( 'NONE',  ( 18.76166303929372603, -2.999999999999992895, -225.1221413045205111 ) ) ;
#19210=DIRECTION ( 'NONE',  ( 0.000000000000000000, 0.000000000000000000, -1.000000000000000000 ) ) ;
#19282=EDGE_LOOP ( 'NONE', ( #21558, #11439, #19934, #9165 ) ) ;
#19343=LINE ( 'NONE', #20697, #10159 ) ;
#19438=EDGE_CURVE ( 'NONE', #9979, #4726, #19343, .T. ) ;
#19455=VECTOR ( 'NONE', #12118, 1000.000000000000000 ) ;
#19527=VECTOR ( 'NONE', #5025, 1000.000000000000000 ) ;
#19543=DIRECTION ( 'NONE',  ( -2.891205793294678696E-17, 0.000000000000000000, -1.000000000000000000 ) ) ;
#19552=EDGE_CURVE ( 'NONE', #18785, #17015, #19838, .T. ) ;
#19586=CARTESIAN_POINT ( 'NONE',  ( 20.79630060232323174, 1.171431775223809035, -222.2327692698370356 ) ) ;
#19604=AXIS2_PLACEMENT_3D ( 'NONE', #247, #10268, #3830 ) ;
#19625=AXIS2_PLACEMENT_3D ( 'NONE', #10884, #748, #19210 ) ;
#19654=ORIENTED_EDGE ( 'NONE', *, *, #7567, .F. ) ;
#19694=CARTESIAN_POINT ( 'NONE',  ( 18.77038210872052559, 2.992569296362963538, -224.7568172542696914 ) ) ;
#19700=AXIS2_PLACEMENT_3D ( 'NONE', #19951, #12777, #7715 ) ;
#19801=CARTESIAN_POINT ( 'NONE',  ( 18.80464855560519055, 2.963306505625483922, -224.5168608946970323 ) ) ;
#19838=CIRCLE ( 'NONE', #17712, 2.000000000000000000 ) ;
#19869=CARTESIAN_POINT ( 'NONE',  ( 2.999999999999971578, 3.673940397442062826E-16, -221.9999999999999716 ) ) ;
#19924=STYLED_ITEM ( 'NONE', ( #12435 ), #14254 ) ;
#19934=ORIENTED_EDGE ( 'NONE', *, *, #21643, .T. ) ;
#19951=CARTESIAN_POINT ( 'NONE',  ( 0.000000000000000000, 0.000000000000000000, -105.0000000000000142 ) ) ;
#19957=VECTOR ( 'NONE', #21493, 1000.000000000000000 ) ;
#19966=DIRECTION ( 'NONE',  ( -1.000000000000000000, 0.000000000000000000, 2.891205793294678696E-17 ) ) ;
#19989=UNCERTAINTY_MEASURE_WITH_UNIT (LENGTH_MEASURE( 1.000000000000000082E-05 ), #1634, 'distance_accuracy_value', 'NONE');
#20000=FACE_OUTER_BOUND ( 'NONE', #5007, .T. ) ;
#20027=DIRECTION ( 'NONE',  ( 0.000000000000000000, 0.000000000000000000, 1.000000000000000000 ) ) ;
#20074=CARTESIAN_POINT ( 'NONE',  ( -6.938893903907228378E-15, 0.000000000000000000, -224.9999999999999716 ) ) ;
#20088=DIRECTION ( 'NONE',  ( 1.000000000000000000, 0.000000000000000000, 0.000000000000000000 ) ) ;
#20099=CARTESIAN_POINT ( 'NONE',  ( 19.38184807124232378, -2.462809743167423626, -223.2754647498610154 ) ) ;
#20104=CARTESIAN_POINT ( 'NONE',  ( 0.000000000000000000, 0.000000000000000000, -120.0000000000000142 ) ) ;
#20145=ORIENTED_EDGE ( 'NONE', *, *, #7567, .T. ) ;
#20209=CARTESIAN_POINT ( 'NONE',  ( 18.76166303929371537, -3.000000000000002665, -225.0000000000001990 ) ) ;
#20213=DIRECTION ( 'NONE',  ( 1.000000000000000000, 0.000000000000000000, 0.000000000000000000 ) ) ;
#20224=CIRCLE ( 'NONE', #16648, 3.000000000000002665 ) ;
#20231=ADVANCED_FACE ( 'NONE', ( #20000 ), #10523, .T. ) ;
#20244=CARTESIAN_POINT ( 'NONE',  ( 18.76166303929371537, -3.000000000000002665, -225.0000000000001990 ) ) ;
#20293=LINE ( 'NONE', #18298, #19198 ) ;
#20321=CARTESIAN_POINT ( 'NONE',  ( -2.000000000000000000, 2.449293598294706414E-16, -105.0000000000000142 ) ) ;
#20328=CARTESIAN_POINT ( 'NONE',  ( 21.91438441781873081, -0.08560050869741445134, -228.0000000000000000 ) ) ;
#20353=PRODUCT_DEFINITION_SHAPE ( 'NONE', 'NONE',  #16346 ) ;
#20357=LINE ( 'NONE', #6648, #4175 ) ;
#20437=CARTESIAN_POINT ( 'NONE',  ( 21.65323058444409909, -0.3442074641359690323, -222.0185703855663348 ) ) ;
#20441=CARTESIAN_POINT ( 'NONE',  ( 20.62542899963628784, -1.332263963074644231, -227.6939020710331363 ) ) ;
#20468=DIRECTION ( 'NONE',  ( 1.000000000000000000, 0.000000000000000000, 0.000000000000000000 ) ) ;
#20576=CARTESIAN_POINT ( 'NONE',  ( 2.999999999999975131, 3.673940397442065291E-16, -105.0000000000000142 ) ) ;
#20697=CARTESIAN_POINT ( 'NONE',  ( 1.322875655532295358, 1.500000000000000000, -104.9999999999999858 ) ) ;
#20710=DIRECTION ( 'NONE',  ( 1.000000000000000000, 0.000000000000000000, 0.000000000000000000 ) ) ;
#20776=CARTESIAN_POINT ( 'NONE',  ( 18.92955364685788666, -2.856280672885344263, -225.9473756571962042 ) ) ;
#20787=ORIENTED_EDGE ( 'NONE', *, *, #8177, .T. ) ;
#20795=( BOUNDED_CURVE ( )  B_SPLINE_CURVE ( 3, ( #21938, #6529, #13399, #17426 ),
 .UNSPECIFIED., .F., .F. ) 
 B_SPLINE_CURVE_WITH_KNOTS ( ( 4, 4 ),
 ( 3.141592653589793116, 6.283185307179586232 ),
 .UNSPECIFIED. ) 
 CURVE ( )  GEOMETRIC_REPRESENTATION_ITEM ( )  RATIONAL_B_SPLINE_CURVE ( ( 1.000000000000000000, 0.3333333333333333703, 0.3333333333333333703, 1.000000000000000000 ) ) 
 REPRESENTATION_ITEM ( '' )  );
#20807=EDGE_CURVE ( 'NONE', #18785, #7031, #15928, .T. ) ;
#20980=ORIENTED_EDGE ( 'NONE', *, *, #7917, .T. ) ;
#20993=AXIS2_PLACEMENT_3D ( 'NONE', #6130, #11320, #16386 ) ;
#21002=CARTESIAN_POINT ( 'NONE',  ( 19.02418198972958407, -2.774848290582036636, -226.1609295929775669 ) ) ;
#21055=STYLED_ITEM ( 'NONE', ( #3371 ), #7772 ) ;
#21123=EDGE_LOOP ( 'NONE', ( #1673, #5881, #6941, #5234 ) ) ;
#21305=VERTEX_POINT ( 'NONE', #8149 ) ;
#21328=DIRECTION ( 'NONE',  ( -2.891205793294678696E-17, 0.000000000000000000, -1.000000000000000000 ) ) ;
#21336=CARTESIAN_POINT ( 'NONE',  ( -3.000000000000033751, 0.000000000000000000, -227.9999999999999716 ) ) ;
#21351=EDGE_CURVE ( 'NONE', #11981, #17126, #10266, .T. ) ;
#21385=CARTESIAN_POINT ( 'NONE',  ( 21.13757381859901940, 0.8461838617116986816, -222.1166354392582889 ) ) ;
#21493=DIRECTION ( 'NONE',  ( -2.891205793294678696E-17, 0.000000000000000000, -1.000000000000000000 ) ) ;
#21558=ORIENTED_EDGE ( 'NONE', *, *, #17379, .F. ) ;
#21601=CARTESIAN_POINT ( 'NONE',  ( 19.25067847059919401, 2.577822808762952000, -223.4500418966247253 ) ) ;
#21643=EDGE_CURVE ( 'NONE', #7031, #4726, #8259, .T. ) ;
#21757=PLANE ( 'NONE',  #29 ) ;
#21797=CARTESIAN_POINT ( 'NONE',  ( 18.76166303929371182, -3.000000000000011990, -224.8780544821428578 ) ) ;
#21829=CARTESIAN_POINT ( 'NONE',  ( 18.93769218002320898, 2.849225658158390573, -225.9458950196911076 ) ) ;
#21854=CARTESIAN_POINT ( 'NONE',  ( 0.000000000000000000, 0.000000000000000000, -105.0000000000000142 ) ) ;
#21938=CARTESIAN_POINT ( 'NONE',  ( 2.999999999999971578, 3.673940397442062826E-16, -221.9999999999999716 ) ) ;
#21940=SURFACE_STYLE_USAGE ( .BOTH. , #11601 ) ;
#21945=ORIENTED_EDGE ( 'NONE', *, *, #9938, .F. ) ;
#21949=CARTESIAN_POINT ( 'NONE',  ( -3.000000000000033751, 0.000000000000000000, -227.9999999999999716 ) ) ;
#22059=CARTESIAN_POINT ( 'NONE',  ( 22.00000000000000000, 6.162975822039154730E-30, -228.0000000000000000 ) ) ;
#22147=CARTESIAN_POINT ( 'NONE',  ( 21.65362371779453454, -0.3438195010044712285, -227.9814669592245195 ) ) ;
#22180=EDGE_LOOP ( 'NONE', ( #6327, #5035, #2086, #13609 ) ) ;
#22261=CARTESIAN_POINT ( 'NONE',  ( -6.938893903907228378E-15, 0.000000000000000000, -224.9999999999999716 ) ) ;
#22265=CARTESIAN_POINT ( 'NONE',  ( -6.938893903907228378E-15, 0.000000000000000000, -224.9999999999999716 ) ) ;
ENDSEC;
END-ISO-10303-21;
